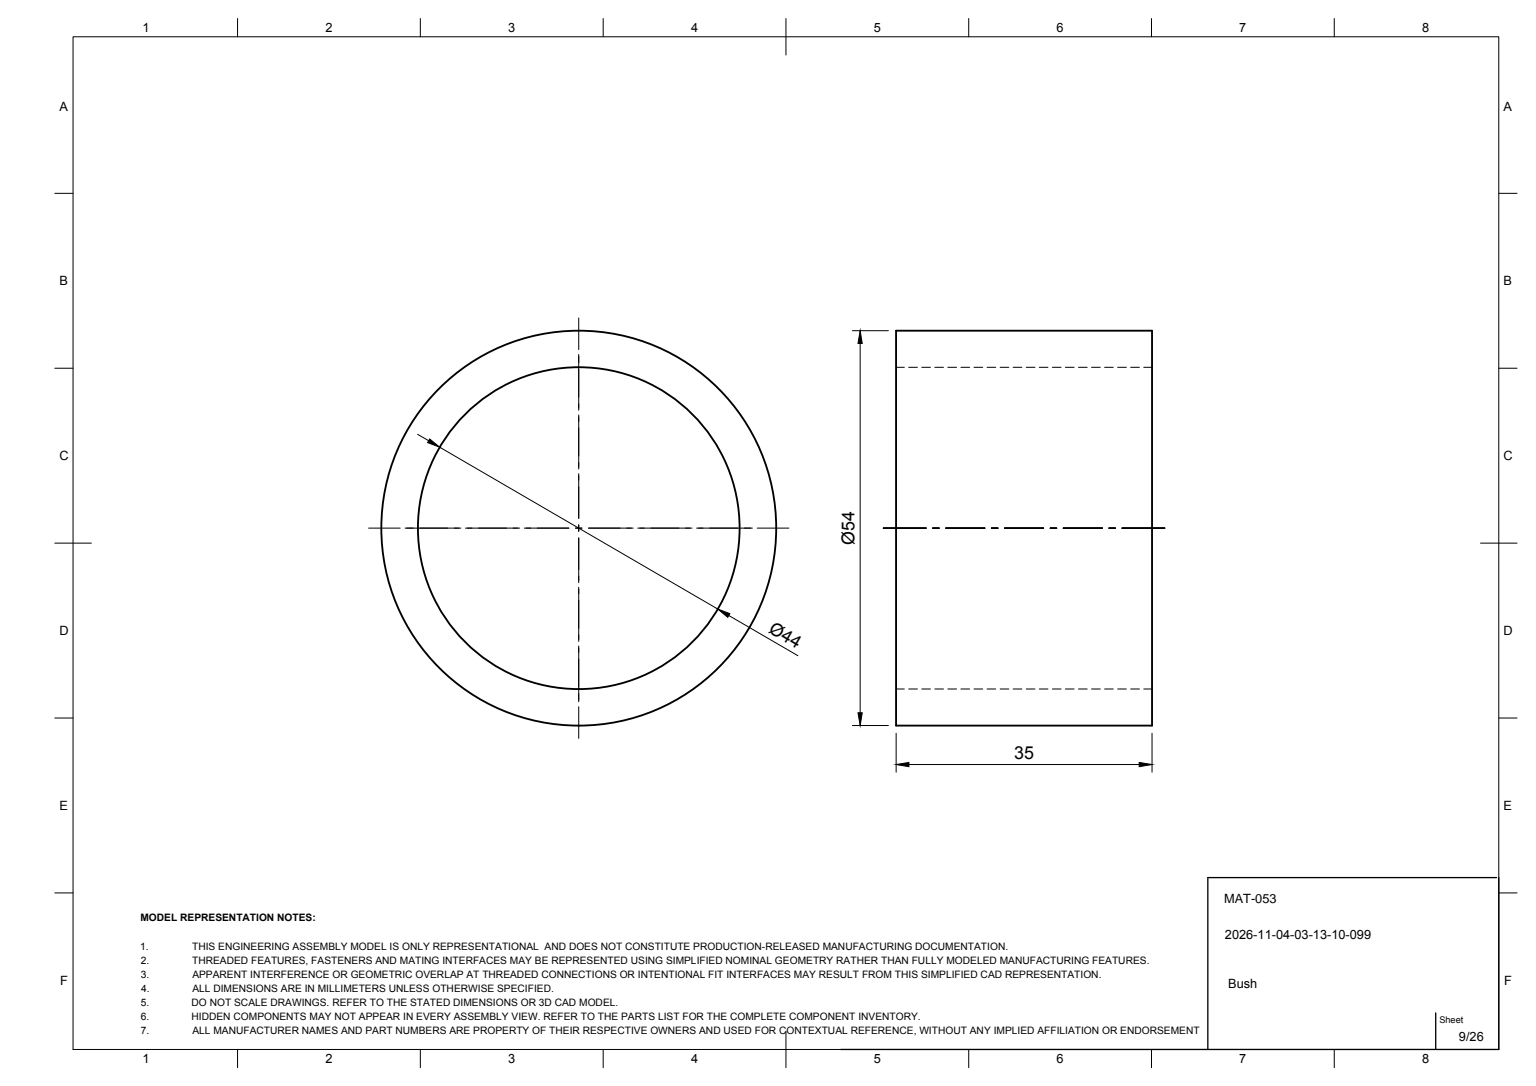
ISO-10303-21;
HEADER;
FILE_DESCRIPTION (('STEP AP214'),
    '1' );
FILE_NAME ('Bush.step',
    '2026-10-10T03:43:58',
    ( '' ),
    ( '' ),
    'SwSTEP 2.0',
    'SolidWorks 2026',
    '' );
FILE_SCHEMA (( 'AUTOMOTIVE_DESIGN' ));
ENDSEC;

DATA;
#284=CARTESIAN_POINT ( 'NONE',  ( 0.000000000000000000, 0.000000000000000000, 0.000000000000000000 ) ) ;
#1287=AXIS2_PLACEMENT_3D ( 'NONE', #68840, #30886, #67483 ) ;
#1599=DIRECTION ( 'NONE',  ( 0.000000000000000000, 1.000000000000000000, 0.000000000000000000 ) ) ;
#1877=PRODUCT_DEFINITION_SHAPE ( 'NONE', 'NONE',  #58964 ) ;
#1961=EDGE_LOOP ( 'NONE', ( #40526, #24326, #2830, #6923 ) ) ;
#2830=ORIENTED_EDGE ( 'NONE', *, *, #17150, .T. ) ;
#3401=CARTESIAN_POINT ( 'NONE',  ( 0.000000000000000000, 0.000000000000000000, -22.00000000000000355 ) ) ;
#3434=EDGE_LOOP ( 'NONE', ( #30327, #19426, #55519, #42432 ) ) ;
#3666=CARTESIAN_POINT ( 'NONE',  ( 0.000000000000000000, 0.000000000000000000, -27.00000000000000000 ) ) ;
#4091=LINE ( 'NONE', #42405, #16612 ) ;
#4272=DIRECTION ( 'NONE',  ( 0.000000000000000000, 0.000000000000000000, -1.000000000000000000 ) ) ;
#4626=ORIENTED_EDGE ( 'NONE', *, *, #17150, .F. ) ;
#5230=CIRCLE ( 'NONE', #44555, 22.00000000000000355 ) ;
#5682=CARTESIAN_POINT ( 'NONE',  ( 0.000000000000000000, 35.00000000000000000, -22.00000000000000355 ) ) ;
#6281=PRODUCT_DEFINITION_FORMATION_WITH_SPECIFIED_SOURCE ( 'ANY', '', #66481, .NOT_KNOWN. ) ;
#6469=ORIENTED_EDGE ( 'NONE', *, *, #66181, .T. ) ;
#6908=( GEOMETRIC_REPRESENTATION_CONTEXT ( 3 ) GLOBAL_UNCERTAINTY_ASSIGNED_CONTEXT ( ( #62733 ) ) GLOBAL_UNIT_ASSIGNED_CONTEXT ( ( #68183, #44094, #12455 ) ) REPRESENTATION_CONTEXT ( 'NONE', 'WORKASPACE' ) );
#6915=ADVANCED_FACE ( 'NONE', ( #28326, #45549 ), #67035, .T. ) ;
#6923=ORIENTED_EDGE ( 'NONE', *, *, #62743, .F. ) ;
#7562=ADVANCED_FACE ( 'NONE', ( #29056 ), #56119, .T. ) ;
#8013=STYLED_ITEM ( 'NONE', ( #62553 ), #17204 ) ;
#8058=DIRECTION ( 'NONE',  ( 0.000000000000000000, 0.000000000000000000, 1.000000000000000000 ) ) ;
#8306=CIRCLE ( 'NONE', #16167, 22.00000000000000355 ) ;
#8319=DIRECTION ( 'NONE',  ( 1.000000000000000000, 0.000000000000000000, 0.000000000000000000 ) ) ;
#9522=DIRECTION ( 'NONE',  ( -0.000000000000000000, -1.000000000000000000, -0.000000000000000000 ) ) ;
#9896=FACE_OUTER_BOUND ( 'NONE', #1961, .T. ) ;
#10537=CARTESIAN_POINT ( 'NONE',  ( 0.000000000000000000, 35.00000000000000000, 0.000000000000000000 ) ) ;
#12415=CIRCLE ( 'NONE', #16862, 27.00000000000000000 ) ;
#12455=( NAMED_UNIT ( * ) SI_UNIT ( $, .STERADIAN. ) SOLID_ANGLE_UNIT ( ) );
#12537=MECHANICAL_DESIGN_GEOMETRIC_PRESENTATION_REPRESENTATION('',(#8013),#6908);
#13348=CARTESIAN_POINT ( 'NONE',  ( 0.000000000000000000, 0.000000000000000000, 0.000000000000000000 ) ) ;
#13670=CYLINDRICAL_SURFACE ( 'NONE', #57633, 22.00000000000000355 ) ;
#13884=LINE ( 'NONE', #51183, #35679 ) ;
#14641=VERTEX_POINT ( 'NONE', #28266 ) ;
#15678=EDGE_LOOP ( 'NONE', ( #19362, #4626 ) ) ;
#15771=ORIENTED_EDGE ( 'NONE', *, *, #61774, .T. ) ;
#16167=AXIS2_PLACEMENT_3D ( 'NONE', #27532, #44053, #55664 ) ;
#16612=VECTOR ( 'NONE', #69121, 1000.000000000000000 ) ;
#16862=AXIS2_PLACEMENT_3D ( 'NONE', #34998, #29716, #68052 ) ;
#17012=EDGE_LOOP ( 'NONE', ( #19883, #40202 ) ) ;
#17150=EDGE_CURVE ( 'NONE', #61608, #62240, #54025, .T. ) ;
#17204=MANIFOLD_SOLID_BREP ( 'Boss-Extrude1', #30577 ) ;
#17527=AXIS2_PLACEMENT_3D ( 'NONE', #64127, #58841, #48968 ) ;
#18607=DIRECTION ( 'NONE',  ( 0.000000000000000000, 0.000000000000000000, -1.000000000000000000 ) ) ;
#18699=AXIS2_PLACEMENT_3D ( 'NONE', #10537, #9522, #58384 ) ;
#18824=DIRECTION ( 'NONE',  ( 0.000000000000000000, -0.000000000000000000, 1.000000000000000000 ) ) ;
#18980=ORIENTED_EDGE ( 'NONE', *, *, #62743, .T. ) ;
#19300=DIRECTION ( 'NONE',  ( 0.000000000000000000, 1.000000000000000000, 0.000000000000000000 ) ) ;
#19362=ORIENTED_EDGE ( 'NONE', *, *, #66181, .F. ) ;
#19426=ORIENTED_EDGE ( 'NONE', *, *, #59193, .T. ) ;
#19649=LINE ( 'NONE', #41462, #46409 ) ;
#19711=AXIS2_PLACEMENT_3D ( 'NONE', #29387, #50498, #66356 ) ;
#19883=ORIENTED_EDGE ( 'NONE', *, *, #41977, .T. ) ;
#20530=EDGE_LOOP ( 'NONE', ( #38873, #49255 ) ) ;
#21103=CIRCLE ( 'NONE', #50326, 22.00000000000000355 ) ;
#22184=SHAPE_REPRESENTATION ( 'Bush', ( #66832 ), #24189 ) ;
#22794=FACE_OUTER_BOUND ( 'NONE', #15678, .T. ) ;
#23150=DIRECTION ( 'NONE',  ( 0.000000000000000000, -0.000000000000000000, 1.000000000000000000 ) ) ;
#23376=APPLICATION_CONTEXT ( 'automotive_design' ) ;
#23622=AXIS2_PLACEMENT_3D ( 'NONE', #43869, #52778, #4272 ) ;
#24189=( GEOMETRIC_REPRESENTATION_CONTEXT ( 3 ) GLOBAL_UNCERTAINTY_ASSIGNED_CONTEXT ( ( #63421 ) ) GLOBAL_UNIT_ASSIGNED_CONTEXT ( ( #46277, #52925, #69458 ) ) REPRESENTATION_CONTEXT ( 'NONE', 'WORKASPACE' ) );
#24283=CIRCLE ( 'NONE', #17527, 27.00000000000000000 ) ;
#24326=ORIENTED_EDGE ( 'NONE', *, *, #54042, .T. ) ;
#25266=VERTEX_POINT ( 'NONE', #48955 ) ;
#25393=DIRECTION ( 'NONE',  ( 0.000000000000000000, 0.000000000000000000, 1.000000000000000000 ) ) ;
#25504=ORIENTED_EDGE ( 'NONE', *, *, #61774, .F. ) ;
#26126=PRODUCT_DEFINITION_CONTEXT ( 'detailed design', #23376, 'design' ) ;
#26299=EDGE_CURVE ( 'NONE', #14641, #41303, #24283, .T. ) ;
#26909=SHAPE_DEFINITION_REPRESENTATION ( #1877, #22184 ) ;
#27021=DIRECTION ( 'NONE',  ( 0.000000000000000000, 1.000000000000000000, 0.000000000000000000 ) ) ;
#27379=CARTESIAN_POINT ( 'NONE',  ( 2.694222958124177204E-15, 35.00000000000000000, 22.00000000000000355 ) ) ;
#27532=CARTESIAN_POINT ( 'NONE',  ( 0.000000000000000000, 0.000000000000000000, 0.000000000000000000 ) ) ;
#27875=AXIS2_PLACEMENT_3D ( 'NONE', #43026, #43379, #59897 ) ;
#28266=CARTESIAN_POINT ( 'NONE',  ( 0.000000000000000000, 35.00000000000000000, -27.00000000000000000 ) ) ;
#28326=FACE_OUTER_BOUND ( 'NONE', #20530, .T. ) ;
#28720=ORIENTED_EDGE ( 'NONE', *, *, #54042, .F. ) ;
#29056=FACE_OUTER_BOUND ( 'NONE', #55556, .T. ) ;
#29072=ADVANCED_FACE ( 'NONE', ( #53441 ), #52754, .F. ) ;
#29387=CARTESIAN_POINT ( 'NONE',  ( 0.000000000000000000, 35.00000000000000000, 0.000000000000000000 ) ) ;
#29716=DIRECTION ( 'NONE',  ( 0.000000000000000000, 1.000000000000000000, 0.000000000000000000 ) ) ;
#30155=CIRCLE ( 'NONE', #27875, 27.00000000000000000 ) ;
#30327=ORIENTED_EDGE ( 'NONE', *, *, #31131, .F. ) ;
#30577=CLOSED_SHELL ( 'NONE', ( #29072, #65700, #6915, #67215, #7562, #53173 ) ) ;
#30751=EDGE_CURVE ( 'NONE', #25266, #64727, #21103, .T. ) ;
#30886=DIRECTION ( 'NONE',  ( 0.000000000000000000, 1.000000000000000000, 0.000000000000000000 ) ) ;
#30893=FACE_OUTER_BOUND ( 'NONE', #3434, .T. ) ;
#31131=EDGE_CURVE ( 'NONE', #64093, #25266, #4091, .T. ) ;
#31493=SHAPE_REPRESENTATION_RELATIONSHIP ( 'NONE' , 'NONE' ,  #22184, #38232 ) ;
#32882=PRODUCT_CONTEXT ( 'NONE', #49323, 'mechanical' ) ;
#33795=EDGE_LOOP ( 'NONE', ( #25504, #53996 ) ) ;
#34998=CARTESIAN_POINT ( 'NONE',  ( 0.000000000000000000, 0.000000000000000000, 0.000000000000000000 ) ) ;
#35326=VECTOR ( 'NONE', #49280, 1000.000000000000000 ) ;
#35679=VECTOR ( 'NONE', #45900, 1000.000000000000000 ) ;
#38232=ADVANCED_BREP_SHAPE_REPRESENTATION ( '', ( #17204, #66832 ), #24189 ) ;
#38873=ORIENTED_EDGE ( 'NONE', *, *, #26299, .T. ) ;
#38984=PLANE ( 'NONE',  #49823 ) ;
#39821=CARTESIAN_POINT ( 'NONE',  ( 3.306546357697853733E-15, 0.000000000000000000, 27.00000000000000000 ) ) ;
#40202=ORIENTED_EDGE ( 'NONE', *, *, #30751, .T. ) ;
#40526=ORIENTED_EDGE ( 'NONE', *, *, #63643, .F. ) ;
#41092=SURFACE_STYLE_USAGE ( .BOTH. , #46352 ) ;
#41303=VERTEX_POINT ( 'NONE', #48672 ) ;
#41462=CARTESIAN_POINT ( 'NONE',  ( 3.306546357697853733E-15, 35.00000000000000000, 27.00000000000000000 ) ) ;
#41977=EDGE_CURVE ( 'NONE', #64727, #25266, #8306, .T. ) ;
#42122=FILL_AREA_STYLE ('',( #56931 ) ) ;
#42405=CARTESIAN_POINT ( 'NONE',  ( 2.694222958124177204E-15, 35.00000000000000000, 22.00000000000000355 ) ) ;
#42432=ORIENTED_EDGE ( 'NONE', *, *, #30751, .F. ) ;
#43026=CARTESIAN_POINT ( 'NONE',  ( 0.000000000000000000, 35.00000000000000000, 0.000000000000000000 ) ) ;
#43270=CIRCLE ( 'NONE', #56763, 22.00000000000000355 ) ;
#43379=DIRECTION ( 'NONE',  ( 0.000000000000000000, 1.000000000000000000, 0.000000000000000000 ) ) ;
#43646=DIRECTION ( 'NONE',  ( 0.000000000000000000, 1.000000000000000000, 0.000000000000000000 ) ) ;
#43869=CARTESIAN_POINT ( 'NONE',  ( 0.000000000000000000, 35.00000000000000000, 0.000000000000000000 ) ) ;
#44053=DIRECTION ( 'NONE',  ( 0.000000000000000000, 1.000000000000000000, 0.000000000000000000 ) ) ;
#44094=( NAMED_UNIT ( * ) PLANE_ANGLE_UNIT ( ) SI_UNIT ( $, .RADIAN. ) );
#44234=FACE_BOUND ( 'NONE', #17012, .T. ) ;
#44555=AXIS2_PLACEMENT_3D ( 'NONE', #67270, #52452, #25393 ) ;
#44558=DIRECTION ( 'NONE',  ( 0.000000000000000000, 0.000000000000000000, 1.000000000000000000 ) ) ;
#45048=CARTESIAN_POINT ( 'NONE',  ( 0.000000000000000000, 35.00000000000000000, 0.000000000000000000 ) ) ;
#45549=FACE_BOUND ( 'NONE', #33795, .T. ) ;
#45900=DIRECTION ( 'NONE',  ( -0.000000000000000000, -1.000000000000000000, -0.000000000000000000 ) ) ;
#46277=( LENGTH_UNIT ( ) NAMED_UNIT ( * ) SI_UNIT ( .MILLI., .METRE. ) );
#46352=SURFACE_SIDE_STYLE ('',( #51649 ) ) ;
#46359=DIRECTION ( 'NONE',  ( -0.000000000000000000, -1.000000000000000000, -0.000000000000000000 ) ) ;
#46409=VECTOR ( 'NONE', #62915, 1000.000000000000000 ) ;
#48235=LINE ( 'NONE', #5682, #35326 ) ;
#48672=CARTESIAN_POINT ( 'NONE',  ( 3.306546357697853733E-15, 35.00000000000000000, 27.00000000000000000 ) ) ;
#48839=EDGE_LOOP ( 'NONE', ( #15771, #63015, #62559, #65490 ) ) ;
#48955=CARTESIAN_POINT ( 'NONE',  ( 2.694222958124177204E-15, 0.000000000000000000, 22.00000000000000355 ) ) ;
#48968=DIRECTION ( 'NONE',  ( 0.000000000000000000, 0.000000000000000000, 1.000000000000000000 ) ) ;
#49255=ORIENTED_EDGE ( 'NONE', *, *, #63643, .T. ) ;
#49280=DIRECTION ( 'NONE',  ( -0.000000000000000000, -1.000000000000000000, -0.000000000000000000 ) ) ;
#49323=APPLICATION_CONTEXT ( 'automotive_design' ) ;
#49773=CARTESIAN_POINT ( 'NONE',  ( 0.000000000000000000, 35.00000000000000000, 0.000000000000000000 ) ) ;
#49823=AXIS2_PLACEMENT_3D ( 'NONE', #284, #27021, #23150 ) ;
#50326=AXIS2_PLACEMENT_3D ( 'NONE', #13348, #19300, #8058 ) ;
#50498=DIRECTION ( 'NONE',  ( -0.000000000000000000, -1.000000000000000000, -0.000000000000000000 ) ) ;
#50530=CARTESIAN_POINT ( 'NONE',  ( 0.000000000000000000, 0.000000000000000000, 0.000000000000000000 ) ) ;
#51183=CARTESIAN_POINT ( 'NONE',  ( 0.000000000000000000, 35.00000000000000000, -27.00000000000000000 ) ) ;
#51387=VERTEX_POINT ( 'NONE', #59464 ) ;
#51649=SURFACE_STYLE_FILL_AREA ( #42122 ) ;
#52452=DIRECTION ( 'NONE',  ( 0.000000000000000000, 1.000000000000000000, 0.000000000000000000 ) ) ;
#52754=CYLINDRICAL_SURFACE ( 'NONE', #18699, 22.00000000000000355 ) ;
#52778=DIRECTION ( 'NONE',  ( -0.000000000000000000, -1.000000000000000000, -0.000000000000000000 ) ) ;
#52925=( NAMED_UNIT ( * ) PLANE_ANGLE_UNIT ( ) SI_UNIT ( $, .RADIAN. ) );
#53122=CYLINDRICAL_SURFACE ( 'NONE', #23622, 27.00000000000000000 ) ;
#53173=ADVANCED_FACE ( 'NONE', ( #30893 ), #13670, .F. ) ;
#53441=FACE_OUTER_BOUND ( 'NONE', #48839, .T. ) ;
#53996=ORIENTED_EDGE ( 'NONE', *, *, #59193, .F. ) ;
#54025=CIRCLE ( 'NONE', #1287, 27.00000000000000000 ) ;
#54042=EDGE_CURVE ( 'NONE', #41303, #61608, #19649, .T. ) ;
#55519=ORIENTED_EDGE ( 'NONE', *, *, #68652, .T. ) ;
#55556=EDGE_LOOP ( 'NONE', ( #28720, #56893, #18980, #6469 ) ) ;
#55664=DIRECTION ( 'NONE',  ( 0.000000000000000000, 0.000000000000000000, 1.000000000000000000 ) ) ;
#56119=CYLINDRICAL_SURFACE ( 'NONE', #19711, 27.00000000000000000 ) ;
#56581=CARTESIAN_POINT ( 'NONE',  ( 0.000000000000000000, 35.00000000000000000, 0.000000000000000000 ) ) ;
#56763=AXIS2_PLACEMENT_3D ( 'NONE', #45048, #43646, #65123 ) ;
#56893=ORIENTED_EDGE ( 'NONE', *, *, #26299, .F. ) ;
#56931=FILL_AREA_STYLE_COLOUR ( '', #65308 ) ;
#57633=AXIS2_PLACEMENT_3D ( 'NONE', #56581, #46359, #18607 ) ;
#58384=DIRECTION ( 'NONE',  ( 0.000000000000000000, 0.000000000000000000, -1.000000000000000000 ) ) ;
#58841=DIRECTION ( 'NONE',  ( 0.000000000000000000, 1.000000000000000000, 0.000000000000000000 ) ) ;
#58964=PRODUCT_DEFINITION ( 'UNKNOWN', '', #6281, #26126 ) ;
#59193=EDGE_CURVE ( 'NONE', #64093, #51387, #43270, .T. ) ;
#59464=CARTESIAN_POINT ( 'NONE',  ( 0.000000000000000000, 35.00000000000000000, -22.00000000000000355 ) ) ;
#59897=DIRECTION ( 'NONE',  ( 0.000000000000000000, 0.000000000000000000, 1.000000000000000000 ) ) ;
#61608=VERTEX_POINT ( 'NONE', #39821 ) ;
#61774=EDGE_CURVE ( 'NONE', #51387, #64093, #5230, .T. ) ;
#62240=VERTEX_POINT ( 'NONE', #3666 ) ;
#62553=PRESENTATION_STYLE_ASSIGNMENT (( #41092 ) ) ;
#62559=ORIENTED_EDGE ( 'NONE', *, *, #41977, .F. ) ;
#62733=UNCERTAINTY_MEASURE_WITH_UNIT (LENGTH_MEASURE( 1.000000000000000082E-05 ), #68183, 'distance_accuracy_value', 'NONE');
#62743=EDGE_CURVE ( 'NONE', #14641, #62240, #13884, .T. ) ;
#62915=DIRECTION ( 'NONE',  ( -0.000000000000000000, -1.000000000000000000, -0.000000000000000000 ) ) ;
#63015=ORIENTED_EDGE ( 'NONE', *, *, #31131, .T. ) ;
#63421=UNCERTAINTY_MEASURE_WITH_UNIT (LENGTH_MEASURE( 1.000000000000000082E-05 ), #46277, 'distance_accuracy_value', 'NONE');
#63643=EDGE_CURVE ( 'NONE', #41303, #14641, #30155, .T. ) ;
#64093=VERTEX_POINT ( 'NONE', #27379 ) ;
#64127=CARTESIAN_POINT ( 'NONE',  ( 0.000000000000000000, 35.00000000000000000, 0.000000000000000000 ) ) ;
#64727=VERTEX_POINT ( 'NONE', #3401 ) ;
#65123=DIRECTION ( 'NONE',  ( 0.000000000000000000, 0.000000000000000000, 1.000000000000000000 ) ) ;
#65308=COLOUR_RGB ( '',0.7921568627450980005, 0.8196078431372548767, 0.9333333333333333481 ) ;
#65490=ORIENTED_EDGE ( 'NONE', *, *, #68652, .F. ) ;
#65700=ADVANCED_FACE ( 'NONE', ( #9896 ), #53122, .T. ) ;
#66181=EDGE_CURVE ( 'NONE', #62240, #61608, #12415, .T. ) ;
#66356=DIRECTION ( 'NONE',  ( 0.000000000000000000, 0.000000000000000000, -1.000000000000000000 ) ) ;
#66481=PRODUCT ( 'Bush', 'Bush', '', ( #32882 ) ) ;
#66832=AXIS2_PLACEMENT_3D ( 'NONE', #50530, #44558, #8319 ) ;
#66884=AXIS2_PLACEMENT_3D ( 'NONE', #49773, #1599, #18824 ) ;
#67035=PLANE ( 'NONE',  #66884 ) ;
#67215=ADVANCED_FACE ( 'NONE', ( #22794, #44234 ), #38984, .F. ) ;
#67270=CARTESIAN_POINT ( 'NONE',  ( 0.000000000000000000, 35.00000000000000000, 0.000000000000000000 ) ) ;
#67483=DIRECTION ( 'NONE',  ( 0.000000000000000000, 0.000000000000000000, 1.000000000000000000 ) ) ;
#68052=DIRECTION ( 'NONE',  ( 0.000000000000000000, 0.000000000000000000, 1.000000000000000000 ) ) ;
#68183=( LENGTH_UNIT ( ) NAMED_UNIT ( * ) SI_UNIT ( .MILLI., .METRE. ) );
#68652=EDGE_CURVE ( 'NONE', #51387, #64727, #48235, .T. ) ;
#68840=CARTESIAN_POINT ( 'NONE',  ( 0.000000000000000000, 0.000000000000000000, 0.000000000000000000 ) ) ;
#69121=DIRECTION ( 'NONE',  ( -0.000000000000000000, -1.000000000000000000, -0.000000000000000000 ) ) ;
#69458=( NAMED_UNIT ( * ) SI_UNIT ( $, .STERADIAN. ) SOLID_ANGLE_UNIT ( ) );
ENDSEC;
END-ISO-10303-21;
